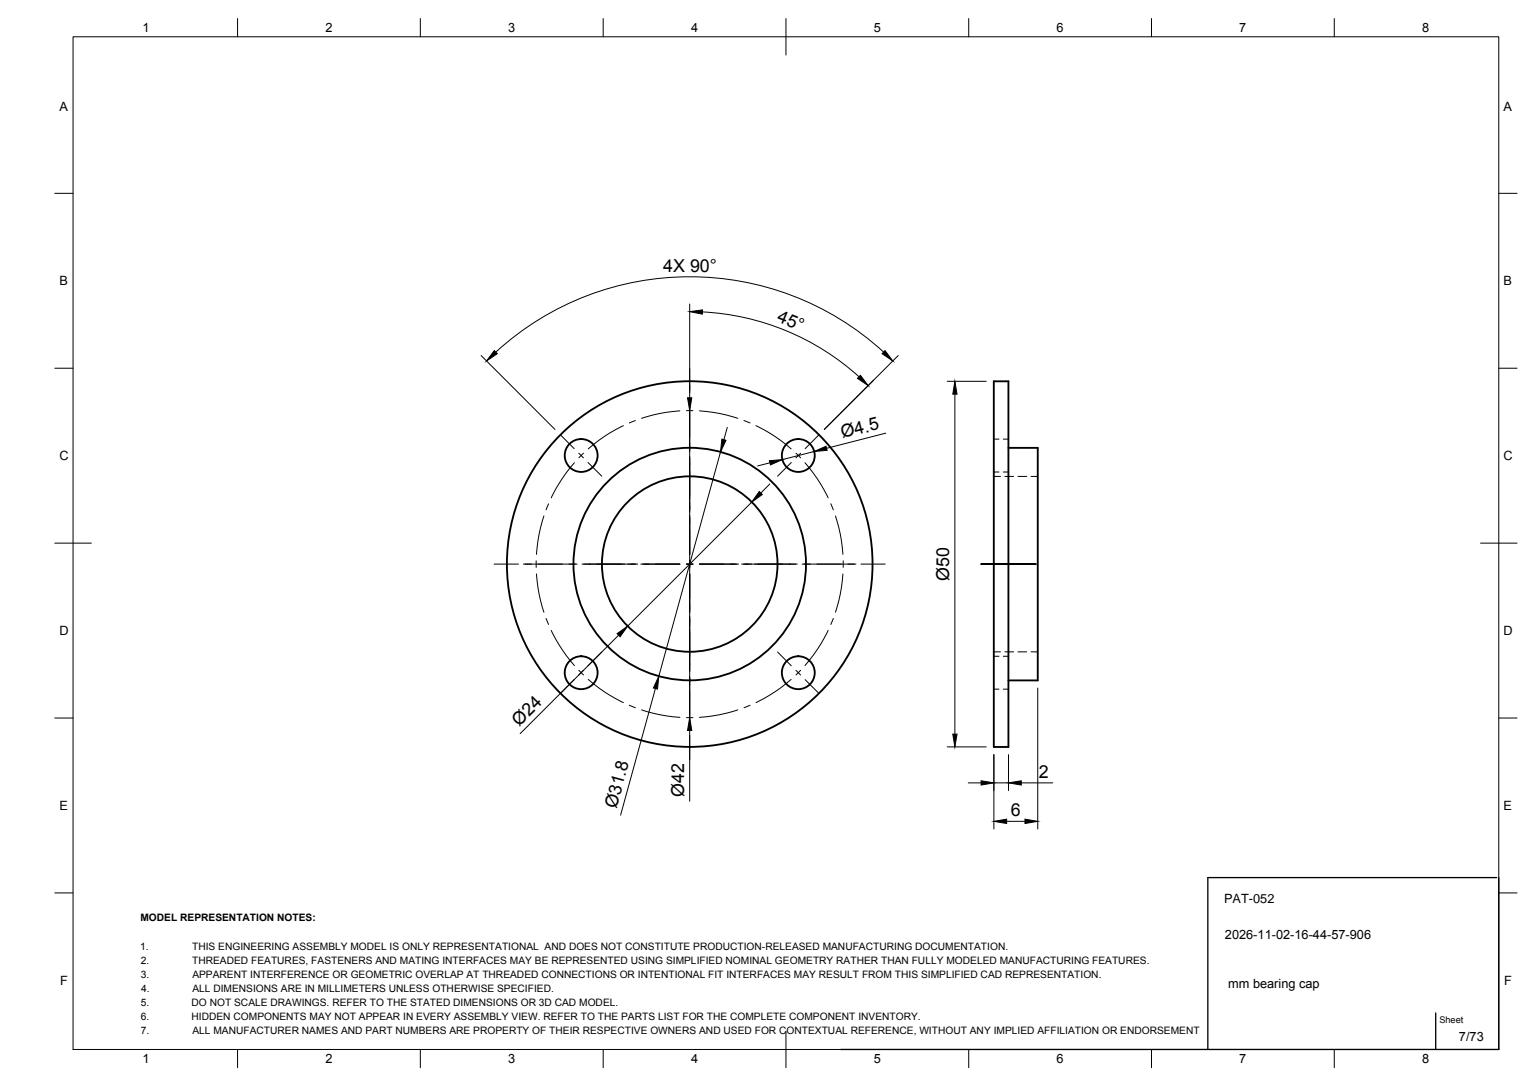
ISO-10303-21;
HEADER;
/* Generated by software containing ST-Developer
 * from STEP Tools, Inc. (www.steptools.com) 
 */

FILE_DESCRIPTION(
/* description */ ('Hand-crank gear train demonstrator'),
/* implementation_level */ '2;1');

FILE_NAME(
/* name */ 'mm bearing cap.step',
/* time_stamp */ '2026-10-28T03:22:13-07:00',
/* author */ (''),
/* organization */ (''),
/* preprocessor_version */ 'ST-DEVELOPER v20.2',
/* originating_system */ 'Autodesk Translation Framework v15.17.0.0',
/* authorisation */ '');

FILE_SCHEMA (('AUTOMOTIVE_DESIGN { 1 0 10303 214 3 1 1 }'));
ENDSEC;

DATA;
#10=MECHANICAL_DESIGN_GEOMETRIC_PRESENTATION_REPRESENTATION('',(#1191),#62758);
#1063=SHAPE_REPRESENTATION_RELATIONSHIP('SRR','None',#63035,#1127);
#1127=ADVANCED_BREP_SHAPE_REPRESENTATION('',(#1270),#62689);
#1191=STYLED_ITEM('',(#63462),#1270);
#1270=MANIFOLD_SOLID_BREP('Body1',#16371);
#1398=FACE_BOUND('',#3163,.T.);
#1399=FACE_BOUND('',#3167,.T.);
#1400=FACE_BOUND('',#3168,.T.);
#1401=FACE_BOUND('',#3169,.T.);
#1402=FACE_BOUND('',#3170,.T.);
#1403=FACE_BOUND('',#3171,.T.);
#1404=FACE_BOUND('',#3173,.T.);
#1405=FACE_BOUND('',#3174,.T.);
#1406=FACE_BOUND('',#3175,.T.);
#1407=FACE_BOUND('',#3176,.T.);
#1408=FACE_BOUND('',#3177,.T.);
#1647=PLANE('',#17276);
#1648=PLANE('',#17283);
#1649=PLANE('',#17284);
#2165=FACE_OUTER_BOUND('',#3157,.T.);
#2166=FACE_OUTER_BOUND('',#3158,.T.);
#2167=FACE_OUTER_BOUND('',#3159,.T.);
#2168=FACE_OUTER_BOUND('',#3160,.T.);
#2169=FACE_OUTER_BOUND('',#3161,.T.);
#2170=FACE_OUTER_BOUND('',#3162,.T.);
#2171=FACE_OUTER_BOUND('',#3164,.T.);
#2172=FACE_OUTER_BOUND('',#3165,.T.);
#2173=FACE_OUTER_BOUND('',#3166,.T.);
#2174=FACE_OUTER_BOUND('',#3172,.T.);
#3157=EDGE_LOOP('',(#11063,#11064,#11065,#11066));
#3158=EDGE_LOOP('',(#11067,#11068,#11069,#11070));
#3159=EDGE_LOOP('',(#11071,#11072,#11073,#11074));
#3160=EDGE_LOOP('',(#11075,#11076,#11077,#11078));
#3161=EDGE_LOOP('',(#11079,#11080,#11081,#11082));
#3162=EDGE_LOOP('',(#11083));
#3163=EDGE_LOOP('',(#11084));
#3164=EDGE_LOOP('',(#11085,#11086,#11087,#11088));
#3165=EDGE_LOOP('',(#11089,#11090,#11091,#11092));
#3166=EDGE_LOOP('',(#11093));
#3167=EDGE_LOOP('',(#11094));
#3168=EDGE_LOOP('',(#11095));
#3169=EDGE_LOOP('',(#11096));
#3170=EDGE_LOOP('',(#11097));
#3171=EDGE_LOOP('',(#11098));
#3172=EDGE_LOOP('',(#11099));
#3173=EDGE_LOOP('',(#11100));
#3174=EDGE_LOOP('',(#11101));
#3175=EDGE_LOOP('',(#11102));
#3176=EDGE_LOOP('',(#11103));
#3177=EDGE_LOOP('',(#11104));
#4344=LINE('',#23550,#5476);
#4345=LINE('',#23556,#5477);
#4346=LINE('',#23562,#5478);
#4347=LINE('',#23568,#5479);
#4348=LINE('',#23574,#5480);
#4349=LINE('',#23581,#5481);
#4350=LINE('',#23587,#5482);
#5476=VECTOR('',#19099,0.225);
#5477=VECTOR('',#19106,0.225);
#5478=VECTOR('',#19113,0.225);
#5479=VECTOR('',#19120,0.225);
#5480=VECTOR('',#19127,1.59);
#5481=VECTOR('',#19136,1.2);
#5482=VECTOR('',#19143,2.5);
#6606=CIRCLE('',#17262,0.225);
#6607=CIRCLE('',#17263,0.225);
#6608=CIRCLE('',#17265,0.225);
#6609=CIRCLE('',#17266,0.225);
#6610=CIRCLE('',#17268,0.225);
#6611=CIRCLE('',#17269,0.225);
#6612=CIRCLE('',#17271,0.225);
#6613=CIRCLE('',#17272,0.225);
#6614=CIRCLE('',#17274,1.59);
#6615=CIRCLE('',#17275,1.59);
#6616=CIRCLE('',#17277,1.2);
#6617=CIRCLE('',#17279,1.2);
#6618=CIRCLE('',#17281,2.5);
#6619=CIRCLE('',#17282,2.5);
#7288=VERTEX_POINT('',#23547);
#7289=VERTEX_POINT('',#23549);
#7290=VERTEX_POINT('',#23553);
#7291=VERTEX_POINT('',#23555);
#7292=VERTEX_POINT('',#23559);
#7293=VERTEX_POINT('',#23561);
#7294=VERTEX_POINT('',#23565);
#7295=VERTEX_POINT('',#23567);
#7296=VERTEX_POINT('',#23571);
#7297=VERTEX_POINT('',#23573);
#7298=VERTEX_POINT('',#23577);
#7299=VERTEX_POINT('',#23580);
#7300=VERTEX_POINT('',#23584);
#7301=VERTEX_POINT('',#23586);
#8783=EDGE_CURVE('',#7288,#7288,#6606,.T.);
#8784=EDGE_CURVE('',#7288,#7289,#4344,.T.);
#8785=EDGE_CURVE('',#7289,#7289,#6607,.T.);
#8786=EDGE_CURVE('',#7290,#7290,#6608,.T.);
#8787=EDGE_CURVE('',#7290,#7291,#4345,.T.);
#8788=EDGE_CURVE('',#7291,#7291,#6609,.T.);
#8789=EDGE_CURVE('',#7292,#7292,#6610,.T.);
#8790=EDGE_CURVE('',#7292,#7293,#4346,.T.);
#8791=EDGE_CURVE('',#7293,#7293,#6611,.T.);
#8792=EDGE_CURVE('',#7294,#7294,#6612,.T.);
#8793=EDGE_CURVE('',#7294,#7295,#4347,.T.);
#8794=EDGE_CURVE('',#7295,#7295,#6613,.T.);
#8795=EDGE_CURVE('',#7296,#7296,#6614,.T.);
#8796=EDGE_CURVE('',#7296,#7297,#4348,.T.);
#8797=EDGE_CURVE('',#7297,#7297,#6615,.T.);
#8798=EDGE_CURVE('',#7298,#7298,#6616,.T.);
#8799=EDGE_CURVE('',#7298,#7299,#4349,.T.);
#8800=EDGE_CURVE('',#7299,#7299,#6617,.T.);
#8801=EDGE_CURVE('',#7300,#7300,#6618,.T.);
#8802=EDGE_CURVE('',#7300,#7301,#4350,.T.);
#8803=EDGE_CURVE('',#7301,#7301,#6619,.T.);
#11063=ORIENTED_EDGE('',*,*,#8783,.F.);
#11064=ORIENTED_EDGE('',*,*,#8784,.T.);
#11065=ORIENTED_EDGE('',*,*,#8785,.F.);
#11066=ORIENTED_EDGE('',*,*,#8784,.F.);
#11067=ORIENTED_EDGE('',*,*,#8786,.F.);
#11068=ORIENTED_EDGE('',*,*,#8787,.T.);
#11069=ORIENTED_EDGE('',*,*,#8788,.F.);
#11070=ORIENTED_EDGE('',*,*,#8787,.F.);
#11071=ORIENTED_EDGE('',*,*,#8789,.F.);
#11072=ORIENTED_EDGE('',*,*,#8790,.T.);
#11073=ORIENTED_EDGE('',*,*,#8791,.F.);
#11074=ORIENTED_EDGE('',*,*,#8790,.F.);
#11075=ORIENTED_EDGE('',*,*,#8792,.F.);
#11076=ORIENTED_EDGE('',*,*,#8793,.T.);
#11077=ORIENTED_EDGE('',*,*,#8794,.F.);
#11078=ORIENTED_EDGE('',*,*,#8793,.F.);
#11079=ORIENTED_EDGE('',*,*,#8795,.F.);
#11080=ORIENTED_EDGE('',*,*,#8796,.T.);
#11081=ORIENTED_EDGE('',*,*,#8797,.F.);
#11082=ORIENTED_EDGE('',*,*,#8796,.F.);
#11083=ORIENTED_EDGE('',*,*,#8795,.T.);
#11084=ORIENTED_EDGE('',*,*,#8798,.T.);
#11085=ORIENTED_EDGE('',*,*,#8798,.F.);
#11086=ORIENTED_EDGE('',*,*,#8799,.T.);
#11087=ORIENTED_EDGE('',*,*,#8800,.T.);
#11088=ORIENTED_EDGE('',*,*,#8799,.F.);
#11089=ORIENTED_EDGE('',*,*,#8801,.F.);
#11090=ORIENTED_EDGE('',*,*,#8802,.T.);
#11091=ORIENTED_EDGE('',*,*,#8803,.T.);
#11092=ORIENTED_EDGE('',*,*,#8802,.F.);
#11093=ORIENTED_EDGE('',*,*,#8801,.T.);
#11094=ORIENTED_EDGE('',*,*,#8797,.T.);
#11095=ORIENTED_EDGE('',*,*,#8794,.T.);
#11096=ORIENTED_EDGE('',*,*,#8791,.T.);
#11097=ORIENTED_EDGE('',*,*,#8788,.T.);
#11098=ORIENTED_EDGE('',*,*,#8785,.T.);
#11099=ORIENTED_EDGE('',*,*,#8803,.F.);
#11100=ORIENTED_EDGE('',*,*,#8800,.F.);
#11101=ORIENTED_EDGE('',*,*,#8792,.T.);
#11102=ORIENTED_EDGE('',*,*,#8789,.T.);
#11103=ORIENTED_EDGE('',*,*,#8786,.T.);
#11104=ORIENTED_EDGE('',*,*,#8783,.T.);
#15195=CYLINDRICAL_SURFACE('',#17261,0.225);
#15196=CYLINDRICAL_SURFACE('',#17264,0.225);
#15197=CYLINDRICAL_SURFACE('',#17267,0.225);
#15198=CYLINDRICAL_SURFACE('',#17270,0.225);
#15199=CYLINDRICAL_SURFACE('',#17273,1.59);
#15200=CYLINDRICAL_SURFACE('',#17278,1.2);
#15201=CYLINDRICAL_SURFACE('',#17280,2.5);
#15475=ADVANCED_FACE('',(#2165),#15195,.F.);
#15476=ADVANCED_FACE('',(#2166),#15196,.F.);
#15477=ADVANCED_FACE('',(#2167),#15197,.F.);
#15478=ADVANCED_FACE('',(#2168),#15198,.F.);
#15479=ADVANCED_FACE('',(#2169),#15199,.T.);
#15480=ADVANCED_FACE('',(#2170,#1398),#1647,.T.);
#15481=ADVANCED_FACE('',(#2171),#15200,.F.);
#15482=ADVANCED_FACE('',(#2172),#15201,.T.);
#15483=ADVANCED_FACE('',(#2173,#1399,#1400,#1401,#1402,#1403),#1648,.T.);
#15484=ADVANCED_FACE('',(#2174,#1404,#1405,#1406,#1407,#1408),#1649,.F.);
#16371=CLOSED_SHELL('',(#15475,#15476,#15477,#15478,#15479,#15480,#15481,
#15482,#15483,#15484));
#17260=AXIS2_PLACEMENT_3D('',#23545,#19093,#19094);
#17261=AXIS2_PLACEMENT_3D('',#23546,#19095,#19096);
#17262=AXIS2_PLACEMENT_3D('',#23548,#19097,#19098);
#17263=AXIS2_PLACEMENT_3D('',#23551,#19100,#19101);
#17264=AXIS2_PLACEMENT_3D('',#23552,#19102,#19103);
#17265=AXIS2_PLACEMENT_3D('',#23554,#19104,#19105);
#17266=AXIS2_PLACEMENT_3D('',#23557,#19107,#19108);
#17267=AXIS2_PLACEMENT_3D('',#23558,#19109,#19110);
#17268=AXIS2_PLACEMENT_3D('',#23560,#19111,#19112);
#17269=AXIS2_PLACEMENT_3D('',#23563,#19114,#19115);
#17270=AXIS2_PLACEMENT_3D('',#23564,#19116,#19117);
#17271=AXIS2_PLACEMENT_3D('',#23566,#19118,#19119);
#17272=AXIS2_PLACEMENT_3D('',#23569,#19121,#19122);
#17273=AXIS2_PLACEMENT_3D('',#23570,#19123,#19124);
#17274=AXIS2_PLACEMENT_3D('',#23572,#19125,#19126);
#17275=AXIS2_PLACEMENT_3D('',#23575,#19128,#19129);
#17276=AXIS2_PLACEMENT_3D('',#23576,#19130,#19131);
#17277=AXIS2_PLACEMENT_3D('',#23578,#19132,#19133);
#17278=AXIS2_PLACEMENT_3D('',#23579,#19134,#19135);
#17279=AXIS2_PLACEMENT_3D('',#23582,#19137,#19138);
#17280=AXIS2_PLACEMENT_3D('',#23583,#19139,#19140);
#17281=AXIS2_PLACEMENT_3D('',#23585,#19141,#19142);
#17282=AXIS2_PLACEMENT_3D('',#23588,#19144,#19145);
#17283=AXIS2_PLACEMENT_3D('',#23589,#19146,#19147);
#17284=AXIS2_PLACEMENT_3D('',#23590,#19148,#19149);
#19093=DIRECTION('axis',(0.,0.,1.));
#19094=DIRECTION('refdir',(1.,0.,0.));
#19095=DIRECTION('center_axis',(0.,1.,0.));
#19096=DIRECTION('ref_axis',(1.,0.,0.));
#19097=DIRECTION('center_axis',(0.,1.,0.));
#19098=DIRECTION('ref_axis',(1.,0.,0.));
#19099=DIRECTION('',(0.,1.,0.));
#19100=DIRECTION('center_axis',(0.,-1.,0.));
#19101=DIRECTION('ref_axis',(1.,0.,0.));
#19102=DIRECTION('center_axis',(0.,1.,0.));
#19103=DIRECTION('ref_axis',(1.,0.,0.));
#19104=DIRECTION('center_axis',(0.,1.,0.));
#19105=DIRECTION('ref_axis',(1.,0.,0.));
#19106=DIRECTION('',(0.,1.,0.));
#19107=DIRECTION('center_axis',(0.,-1.,0.));
#19108=DIRECTION('ref_axis',(1.,0.,0.));
#19109=DIRECTION('center_axis',(0.,1.,0.));
#19110=DIRECTION('ref_axis',(1.,0.,0.));
#19111=DIRECTION('center_axis',(0.,1.,0.));
#19112=DIRECTION('ref_axis',(1.,0.,0.));
#19113=DIRECTION('',(0.,1.,0.));
#19114=DIRECTION('center_axis',(0.,-1.,0.));
#19115=DIRECTION('ref_axis',(1.,0.,0.));
#19116=DIRECTION('center_axis',(0.,1.,0.));
#19117=DIRECTION('ref_axis',(1.,0.,0.));
#19118=DIRECTION('center_axis',(0.,1.,0.));
#19119=DIRECTION('ref_axis',(1.,0.,0.));
#19120=DIRECTION('',(0.,1.,0.));
#19121=DIRECTION('center_axis',(0.,-1.,0.));
#19122=DIRECTION('ref_axis',(1.,0.,0.));
#19123=DIRECTION('center_axis',(0.,1.,0.));
#19124=DIRECTION('ref_axis',(1.,0.,0.));
#19125=DIRECTION('center_axis',(0.,1.,0.));
#19126=DIRECTION('ref_axis',(1.,0.,0.));
#19127=DIRECTION('',(0.,-1.,0.));
#19128=DIRECTION('center_axis',(0.,-1.,0.));
#19129=DIRECTION('ref_axis',(1.,0.,0.));
#19130=DIRECTION('center_axis',(0.,1.,0.));
#19131=DIRECTION('ref_axis',(1.,0.,0.));
#19132=DIRECTION('center_axis',(0.,-1.,0.));
#19133=DIRECTION('ref_axis',(1.,0.,0.));
#19134=DIRECTION('center_axis',(0.,1.,0.));
#19135=DIRECTION('ref_axis',(1.,0.,0.));
#19136=DIRECTION('',(0.,-1.,0.));
#19137=DIRECTION('center_axis',(0.,-1.,0.));
#19138=DIRECTION('ref_axis',(1.,0.,0.));
#19139=DIRECTION('center_axis',(0.,1.,0.));
#19140=DIRECTION('ref_axis',(1.,0.,0.));
#19141=DIRECTION('center_axis',(0.,1.,0.));
#19142=DIRECTION('ref_axis',(1.,0.,0.));
#19143=DIRECTION('',(0.,-1.,0.));
#19144=DIRECTION('center_axis',(0.,1.,0.));
#19145=DIRECTION('ref_axis',(1.,0.,0.));
#19146=DIRECTION('center_axis',(0.,1.,0.));
#19147=DIRECTION('ref_axis',(1.,0.,0.));
#19148=DIRECTION('center_axis',(0.,1.,0.));
#19149=DIRECTION('ref_axis',(1.,0.,0.));
#23545=CARTESIAN_POINT('',(0.,0.,0.));
#23546=CARTESIAN_POINT('Origin',(-1.48492424049175,-2.7,7.51507575950825));
#23547=CARTESIAN_POINT('',(-1.70992424049175,-2.6,7.51507575950825));
#23548=CARTESIAN_POINT('Origin',(-1.48492424049175,-2.6,7.51507575950825));
#23549=CARTESIAN_POINT('',(-1.70992424049175,-2.4,7.51507575950825));
#23550=CARTESIAN_POINT('',(-1.70992424049175,-2.7,7.51507575950825));
#23551=CARTESIAN_POINT('Origin',(-1.48492424049175,-2.4,7.51507575950825));
#23552=CARTESIAN_POINT('Origin',(-1.48492424049175,-2.7,10.4849242404918));
#23553=CARTESIAN_POINT('',(-1.70992424049175,-2.6,10.4849242404918));
#23554=CARTESIAN_POINT('Origin',(-1.48492424049175,-2.6,10.4849242404918));
#23555=CARTESIAN_POINT('',(-1.70992424049175,-2.4,10.4849242404918));
#23556=CARTESIAN_POINT('',(-1.70992424049175,-2.7,10.4849242404918));
#23557=CARTESIAN_POINT('Origin',(-1.48492424049175,-2.4,10.4849242404918));
#23558=CARTESIAN_POINT('Origin',(1.48492424049175,-2.7,10.4849242404918));
#23559=CARTESIAN_POINT('',(1.25992424049175,-2.6,10.4849242404918));
#23560=CARTESIAN_POINT('Origin',(1.48492424049175,-2.6,10.4849242404918));
#23561=CARTESIAN_POINT('',(1.25992424049175,-2.4,10.4849242404918));
#23562=CARTESIAN_POINT('',(1.25992424049175,-2.7,10.4849242404918));
#23563=CARTESIAN_POINT('Origin',(1.48492424049175,-2.4,10.4849242404918));
#23564=CARTESIAN_POINT('Origin',(1.48492424049175,-2.7,7.51507575950825));
#23565=CARTESIAN_POINT('',(1.25992424049175,-2.6,7.51507575950825));
#23566=CARTESIAN_POINT('Origin',(1.48492424049175,-2.6,7.51507575950825));
#23567=CARTESIAN_POINT('',(1.25992424049175,-2.4,7.51507575950825));
#23568=CARTESIAN_POINT('',(1.25992424049175,-2.7,7.51507575950825));
#23569=CARTESIAN_POINT('Origin',(1.48492424049175,-2.4,7.51507575950825));
#23570=CARTESIAN_POINT('Origin',(0.,-2.4,9.));
#23571=CARTESIAN_POINT('',(-1.59,-2.,9.));
#23572=CARTESIAN_POINT('Origin',(0.,-2.,9.));
#23573=CARTESIAN_POINT('',(-1.59,-2.4,9.));
#23574=CARTESIAN_POINT('',(-1.59,-2.4,9.));
#23575=CARTESIAN_POINT('Origin',(0.,-2.4,9.));
#23576=CARTESIAN_POINT('Origin',(0.,-2.,9.));
#23577=CARTESIAN_POINT('',(-1.2,-2.,9.));
#23578=CARTESIAN_POINT('Origin',(0.,-2.,9.));
#23579=CARTESIAN_POINT('Origin',(0.,-2.6,9.));
#23580=CARTESIAN_POINT('',(-1.2,-2.6,9.));
#23581=CARTESIAN_POINT('',(-1.2,-2.6,9.));
#23582=CARTESIAN_POINT('Origin',(0.,-2.6,9.));
#23583=CARTESIAN_POINT('Origin',(0.,-2.6,9.));
#23584=CARTESIAN_POINT('',(-2.5,-2.4,9.));
#23585=CARTESIAN_POINT('Origin',(0.,-2.4,9.));
#23586=CARTESIAN_POINT('',(-2.5,-2.6,9.));
#23587=CARTESIAN_POINT('',(-2.5,-2.6,9.));
#23588=CARTESIAN_POINT('Origin',(0.,-2.6,9.));
#23589=CARTESIAN_POINT('Origin',(0.,-2.4,9.));
#23590=CARTESIAN_POINT('Origin',(0.,-2.6,9.));
#62615=UNCERTAINTY_MEASURE_WITH_UNIT(LENGTH_MEASURE(0.001),#62759,
'DISTANCE_ACCURACY_VALUE',
'Maximum model space distance between geometric entities at asserted c
onnectivities');
#62684=UNCERTAINTY_MEASURE_WITH_UNIT(LENGTH_MEASURE(0.001),#62759,
'DISTANCE_ACCURACY_VALUE',
'Maximum model space distance between geometric entities at asserted c
onnectivities');
#62689=(
GEOMETRIC_REPRESENTATION_CONTEXT(3)
GLOBAL_UNCERTAINTY_ASSIGNED_CONTEXT((#62615))
GLOBAL_UNIT_ASSIGNED_CONTEXT((#62759,#62761,#62762))
REPRESENTATION_CONTEXT('','3D')
);
#62758=(
GEOMETRIC_REPRESENTATION_CONTEXT(3)
GLOBAL_UNCERTAINTY_ASSIGNED_CONTEXT((#62684))
GLOBAL_UNIT_ASSIGNED_CONTEXT((#62759,#62761,#62762))
REPRESENTATION_CONTEXT('','3D')
);
#62759=(
LENGTH_UNIT()
NAMED_UNIT(*)
SI_UNIT(.CENTI.,.METRE.)
);
#62761=(
NAMED_UNIT(*)
PLANE_ANGLE_UNIT()
SI_UNIT($,.RADIAN.)
);
#62762=(
NAMED_UNIT(*)
SI_UNIT($,.STERADIAN.)
SOLID_ANGLE_UNIT()
);
#62767=SHAPE_DEFINITION_REPRESENTATION(#62840,#63035);
#62840=PRODUCT_DEFINITION_SHAPE('',$,#63109);
#63035=SHAPE_REPRESENTATION('',(#17260),#62689);
#63104=PRODUCT_DEFINITION_CONTEXT('part definition',#63325,'design');
#63109=PRODUCT_DEFINITION('mm bearing cap','mm bearing cap',#63182,#63104);
#63182=PRODUCT_DEFINITION_FORMATION('',$,#63331);
#63325=APPLICATION_CONTEXT(
'Core Data for Automotive Mechanical Design Process');
#63326=PRODUCT_CONTEXT('part definition',#63325,'mechanical');
#63331=PRODUCT('mm bearing cap','mm bearing cap','mm bearing cap',(#63326));
#63456=COLOUR_RGB('Grey',0.48,0.52,0.57);
#63457=FILL_AREA_STYLE_COLOUR('',#63456);
#63458=FILL_AREA_STYLE('',(#63457));
#63459=SURFACE_STYLE_FILL_AREA(#63458);
#63460=SURFACE_SIDE_STYLE('',(#63459));
#63461=SURFACE_STYLE_USAGE(.BOTH.,#63460);
#63462=PRESENTATION_STYLE_ASSIGNMENT((#63461));
ENDSEC;
END-ISO-10303-21;
